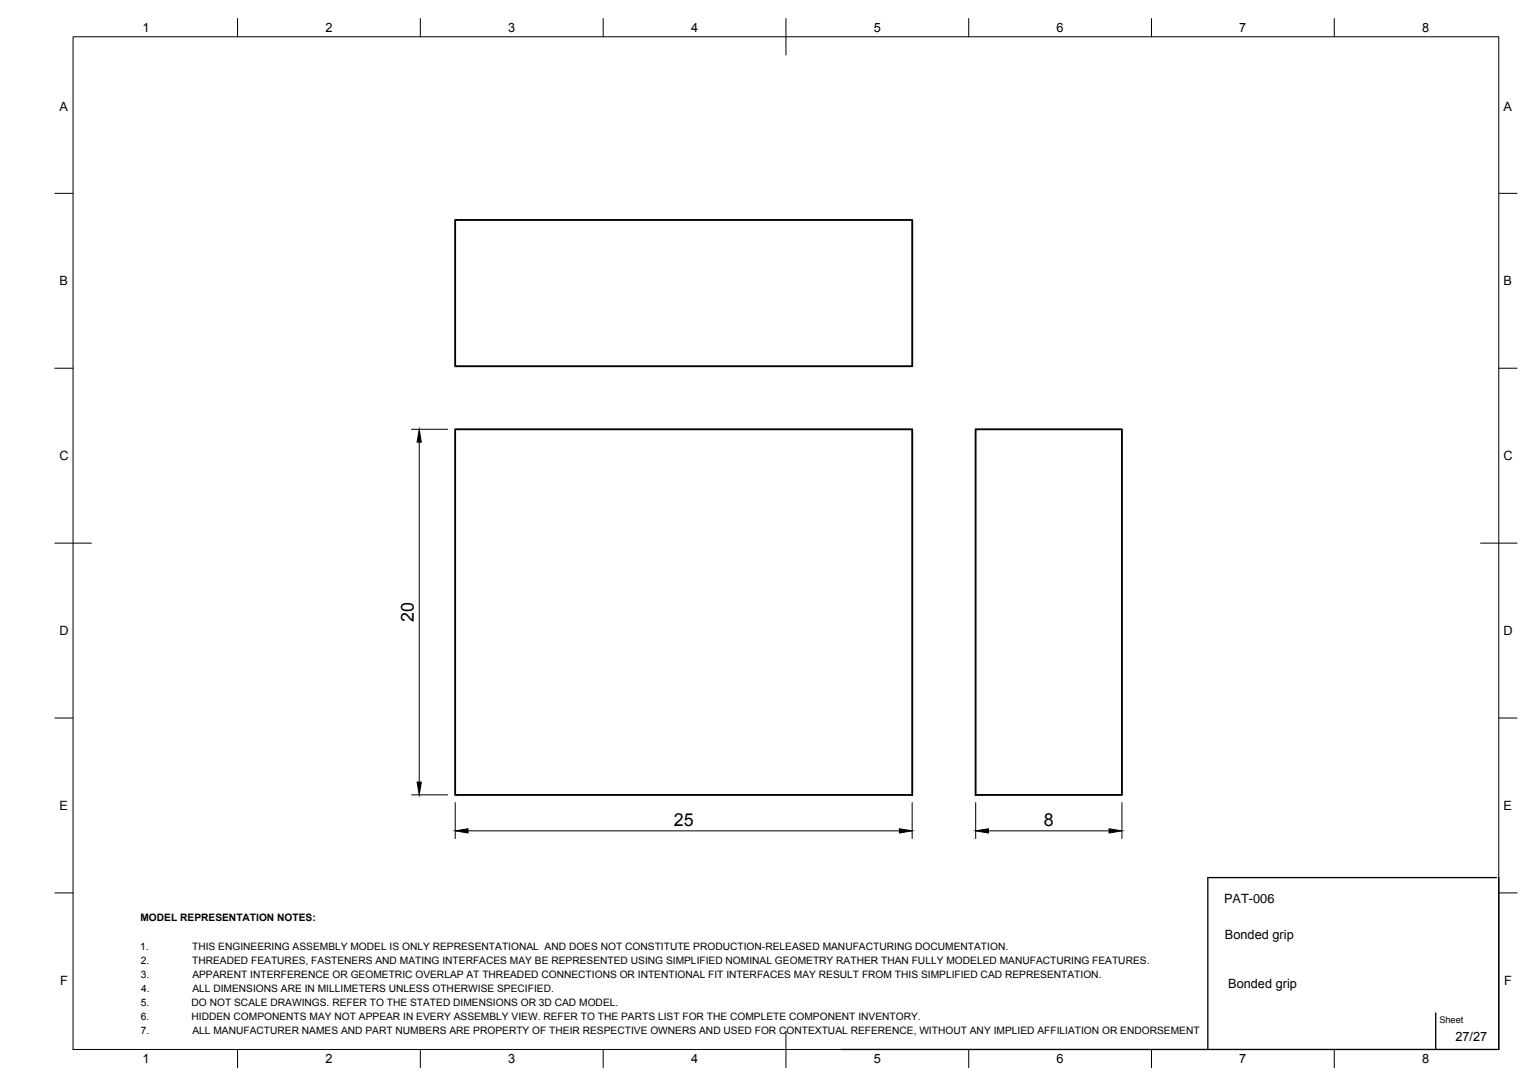
ISO-10303-21;
HEADER;
/* Generated by software containing ST-Developer
 * from STEP Tools, Inc. (www.steptools.com) 
 */

FILE_DESCRIPTION(
/* description */ ('Ball-type isolation valve (generic)'),
/* implementation_level */ '2;1');

FILE_NAME(
/* name */ 'Bonded grip.step',
/* time_stamp */ '2026-10-27T10:53:05-07:00',
/* author */ (''),
/* organization */ (''),
/* preprocessor_version */ 'ST-DEVELOPER v20.2',
/* originating_system */ 'Autodesk Translation Framework v15.17.0.0',
/* authorisation */ '');

FILE_SCHEMA (('AUTOMOTIVE_DESIGN { 1 0 10303 214 3 1 1 }'));
ENDSEC;

DATA;
#10=MECHANICAL_DESIGN_GEOMETRIC_PRESENTATION_REPRESENTATION('',(#301),#7425);
#249=SHAPE_REPRESENTATION_RELATIONSHIP('SRR','None',#7560,#275);
#275=ADVANCED_BREP_SHAPE_REPRESENTATION('',(#325),#7423);
#301=STYLED_ITEM('',(#7751),#325);
#325=MANIFOLD_SOLID_BREP('Body1',#4108);
#562=PLANE('',#4858);
#563=PLANE('',#4859);
#564=PLANE('',#4860);
#565=PLANE('',#4861);
#566=PLANE('',#4862);
#567=PLANE('',#4863);
#806=FACE_OUTER_BOUND('',#1142,.T.);
#807=FACE_OUTER_BOUND('',#1143,.T.);
#808=FACE_OUTER_BOUND('',#1144,.T.);
#809=FACE_OUTER_BOUND('',#1145,.T.);
#810=FACE_OUTER_BOUND('',#1146,.T.);
#811=FACE_OUTER_BOUND('',#1147,.T.);
#1142=EDGE_LOOP('',(#3681,#3682,#3683,#3684));
#1143=EDGE_LOOP('',(#3685,#3686,#3687,#3688));
#1144=EDGE_LOOP('',(#3689,#3690,#3691,#3692));
#1145=EDGE_LOOP('',(#3693,#3694,#3695,#3696));
#1146=EDGE_LOOP('',(#3697,#3698,#3699,#3700));
#1147=EDGE_LOOP('',(#3701,#3702,#3703,#3704));
#1438=LINE('',#7269,#1746);
#1439=LINE('',#7271,#1747);
#1440=LINE('',#7273,#1748);
#1441=LINE('',#7274,#1749);
#1442=LINE('',#7277,#1750);
#1443=LINE('',#7279,#1751);
#1444=LINE('',#7280,#1752);
#1445=LINE('',#7283,#1753);
#1446=LINE('',#7285,#1754);
#1447=LINE('',#7286,#1755);
#1448=LINE('',#7288,#1756);
#1449=LINE('',#7289,#1757);
#1746=VECTOR('',#6091,1.);
#1747=VECTOR('',#6092,1.);
#1748=VECTOR('',#6093,1.);
#1749=VECTOR('',#6094,1.);
#1750=VECTOR('',#6097,1.);
#1751=VECTOR('',#6098,1.);
#1752=VECTOR('',#6099,1.);
#1753=VECTOR('',#6102,1.);
#1754=VECTOR('',#6103,1.);
#1755=VECTOR('',#6104,1.);
#1756=VECTOR('',#6107,1.);
#1757=VECTOR('',#6108,1.);
#2253=VERTEX_POINT('',#7267);
#2254=VERTEX_POINT('',#7268);
#2255=VERTEX_POINT('',#7270);
#2256=VERTEX_POINT('',#7272);
#2257=VERTEX_POINT('',#7276);
#2258=VERTEX_POINT('',#7278);
#2259=VERTEX_POINT('',#7282);
#2260=VERTEX_POINT('',#7284);
#2733=EDGE_CURVE('',#2253,#2254,#1438,.T.);
#2734=EDGE_CURVE('',#2254,#2255,#1439,.T.);
#2735=EDGE_CURVE('',#2256,#2255,#1440,.T.);
#2736=EDGE_CURVE('',#2253,#2256,#1441,.T.);
#2737=EDGE_CURVE('',#2257,#2253,#1442,.T.);
#2738=EDGE_CURVE('',#2258,#2256,#1443,.T.);
#2739=EDGE_CURVE('',#2257,#2258,#1444,.T.);
#2740=EDGE_CURVE('',#2259,#2257,#1445,.T.);
#2741=EDGE_CURVE('',#2260,#2258,#1446,.T.);
#2742=EDGE_CURVE('',#2259,#2260,#1447,.T.);
#2743=EDGE_CURVE('',#2254,#2259,#1448,.T.);
#2744=EDGE_CURVE('',#2255,#2260,#1449,.T.);
#3681=ORIENTED_EDGE('',*,*,#2733,.T.);
#3682=ORIENTED_EDGE('',*,*,#2734,.T.);
#3683=ORIENTED_EDGE('',*,*,#2735,.F.);
#3684=ORIENTED_EDGE('',*,*,#2736,.F.);
#3685=ORIENTED_EDGE('',*,*,#2737,.T.);
#3686=ORIENTED_EDGE('',*,*,#2736,.T.);
#3687=ORIENTED_EDGE('',*,*,#2738,.F.);
#3688=ORIENTED_EDGE('',*,*,#2739,.F.);
#3689=ORIENTED_EDGE('',*,*,#2740,.T.);
#3690=ORIENTED_EDGE('',*,*,#2739,.T.);
#3691=ORIENTED_EDGE('',*,*,#2741,.F.);
#3692=ORIENTED_EDGE('',*,*,#2742,.F.);
#3693=ORIENTED_EDGE('',*,*,#2743,.T.);
#3694=ORIENTED_EDGE('',*,*,#2742,.T.);
#3695=ORIENTED_EDGE('',*,*,#2744,.F.);
#3696=ORIENTED_EDGE('',*,*,#2734,.F.);
#3697=ORIENTED_EDGE('',*,*,#2744,.T.);
#3698=ORIENTED_EDGE('',*,*,#2741,.T.);
#3699=ORIENTED_EDGE('',*,*,#2738,.T.);
#3700=ORIENTED_EDGE('',*,*,#2735,.T.);
#3701=ORIENTED_EDGE('',*,*,#2743,.F.);
#3702=ORIENTED_EDGE('',*,*,#2733,.F.);
#3703=ORIENTED_EDGE('',*,*,#2737,.F.);
#3704=ORIENTED_EDGE('',*,*,#2740,.F.);
#4060=ADVANCED_FACE('',(#806),#562,.T.);
#4061=ADVANCED_FACE('',(#807),#563,.T.);
#4062=ADVANCED_FACE('',(#808),#564,.T.);
#4063=ADVANCED_FACE('',(#809),#565,.T.);
#4064=ADVANCED_FACE('',(#810),#566,.T.);
#4065=ADVANCED_FACE('',(#811),#567,.F.);
#4108=CLOSED_SHELL('',(#4060,#4061,#4062,#4063,#4064,#4065));
#4857=AXIS2_PLACEMENT_3D('',#7265,#6087,#6088);
#4858=AXIS2_PLACEMENT_3D('',#7266,#6089,#6090);
#4859=AXIS2_PLACEMENT_3D('',#7275,#6095,#6096);
#4860=AXIS2_PLACEMENT_3D('',#7281,#6100,#6101);
#4861=AXIS2_PLACEMENT_3D('',#7287,#6105,#6106);
#4862=AXIS2_PLACEMENT_3D('',#7290,#6109,#6110);
#4863=AXIS2_PLACEMENT_3D('',#7291,#6111,#6112);
#6087=DIRECTION('axis',(0.,0.,1.));
#6088=DIRECTION('refdir',(1.,0.,0.));
#6089=DIRECTION('center_axis',(0.,1.,0.));
#6090=DIRECTION('ref_axis',(-1.,0.,0.));
#6091=DIRECTION('',(-1.,0.,0.));
#6092=DIRECTION('',(0.,0.,1.));
#6093=DIRECTION('',(-1.,0.,0.));
#6094=DIRECTION('',(0.,0.,1.));
#6095=DIRECTION('center_axis',(1.,0.,0.));
#6096=DIRECTION('ref_axis',(0.,1.,0.));
#6097=DIRECTION('',(0.,1.,0.));
#6098=DIRECTION('',(0.,1.,0.));
#6099=DIRECTION('',(0.,0.,1.));
#6100=DIRECTION('center_axis',(0.,-1.,0.));
#6101=DIRECTION('ref_axis',(1.,0.,0.));
#6102=DIRECTION('',(1.,0.,0.));
#6103=DIRECTION('',(1.,0.,0.));
#6104=DIRECTION('',(0.,0.,1.));
#6105=DIRECTION('center_axis',(-1.,0.,0.));
#6106=DIRECTION('ref_axis',(0.,-1.,0.));
#6107=DIRECTION('',(0.,-1.,0.));
#6108=DIRECTION('',(0.,-1.,0.));
#6109=DIRECTION('center_axis',(0.,0.,1.));
#6110=DIRECTION('ref_axis',(1.,0.,0.));
#6111=DIRECTION('center_axis',(0.,0.,1.));
#6112=DIRECTION('ref_axis',(1.,0.,0.));
#7265=CARTESIAN_POINT('',(0.,0.,0.));
#7266=CARTESIAN_POINT('Origin',(8.5,1.,9.4));
#7267=CARTESIAN_POINT('',(8.5,1.,9.4));
#7268=CARTESIAN_POINT('',(6.,1.,9.4));
#7269=CARTESIAN_POINT('',(8.5,1.,9.4));
#7270=CARTESIAN_POINT('',(6.,1.,10.2));
#7271=CARTESIAN_POINT('',(6.,1.,9.4));
#7272=CARTESIAN_POINT('',(8.5,1.,10.2));
#7273=CARTESIAN_POINT('',(8.5,1.,10.2));
#7274=CARTESIAN_POINT('',(8.5,1.,9.4));
#7275=CARTESIAN_POINT('Origin',(8.5,-1.,9.4));
#7276=CARTESIAN_POINT('',(8.5,-1.,9.4));
#7277=CARTESIAN_POINT('',(8.5,-1.,9.4));
#7278=CARTESIAN_POINT('',(8.5,-1.,10.2));
#7279=CARTESIAN_POINT('',(8.5,-1.,10.2));
#7280=CARTESIAN_POINT('',(8.5,-1.,9.4));
#7281=CARTESIAN_POINT('Origin',(6.,-1.,9.4));
#7282=CARTESIAN_POINT('',(6.,-1.,9.4));
#7283=CARTESIAN_POINT('',(6.,-1.,9.4));
#7284=CARTESIAN_POINT('',(6.,-1.,10.2));
#7285=CARTESIAN_POINT('',(6.,-1.,10.2));
#7286=CARTESIAN_POINT('',(6.,-1.,9.4));
#7287=CARTESIAN_POINT('Origin',(6.,1.,9.4));
#7288=CARTESIAN_POINT('',(6.,1.,9.4));
#7289=CARTESIAN_POINT('',(6.,1.,10.2));
#7290=CARTESIAN_POINT('Origin',(7.25,0.,10.2));
#7291=CARTESIAN_POINT('Origin',(7.25,0.,9.4));
#7393=UNCERTAINTY_MEASURE_WITH_UNIT(LENGTH_MEASURE(0.001),#7426,
'DISTANCE_ACCURACY_VALUE',
'Maximum model space distance between geometric entities at asserted c
onnectivities');
#7395=UNCERTAINTY_MEASURE_WITH_UNIT(LENGTH_MEASURE(0.001),#7426,
'DISTANCE_ACCURACY_VALUE',
'Maximum model space distance between geometric entities at asserted c
onnectivities');
#7423=(
GEOMETRIC_REPRESENTATION_CONTEXT(3)
GLOBAL_UNCERTAINTY_ASSIGNED_CONTEXT((#7393))
GLOBAL_UNIT_ASSIGNED_CONTEXT((#7426,#7428,#7429))
REPRESENTATION_CONTEXT('','3D')
);
#7425=(
GEOMETRIC_REPRESENTATION_CONTEXT(3)
GLOBAL_UNCERTAINTY_ASSIGNED_CONTEXT((#7395))
GLOBAL_UNIT_ASSIGNED_CONTEXT((#7426,#7428,#7429))
REPRESENTATION_CONTEXT('','3D')
);
#7426=(
LENGTH_UNIT()
NAMED_UNIT(*)
SI_UNIT(.CENTI.,.METRE.)
);
#7428=(
NAMED_UNIT(*)
PLANE_ANGLE_UNIT()
SI_UNIT($,.RADIAN.)
);
#7429=(
NAMED_UNIT(*)
SI_UNIT($,.STERADIAN.)
SOLID_ANGLE_UNIT()
);
#7457=SHAPE_DEFINITION_REPRESENTATION(#7523,#7560);
#7523=PRODUCT_DEFINITION_SHAPE('',$,#7590);
#7560=SHAPE_REPRESENTATION('',(#4857),#7423);
#7562=PRODUCT_DEFINITION_CONTEXT('part definition',#7651,'design');
#7590=PRODUCT_DEFINITION('Bonded grip','Bonded grip',#7619,#7562);
#7619=PRODUCT_DEFINITION_FORMATION('',$,#7680);
#7651=APPLICATION_CONTEXT(
'Core Data for Automotive Mechanical Design Process');
#7652=PRODUCT_CONTEXT('part definition',#7651,'mechanical');
#7680=PRODUCT('Bonded grip','Bonded grip','Bonded grip',(#7652));
#7745=COLOUR_RGB('Black',0.12,0.14,0.17);
#7746=FILL_AREA_STYLE_COLOUR('',#7745);
#7747=FILL_AREA_STYLE('',(#7746));
#7748=SURFACE_STYLE_FILL_AREA(#7747);
#7749=SURFACE_SIDE_STYLE('',(#7748));
#7750=SURFACE_STYLE_USAGE(.BOTH.,#7749);
#7751=PRESENTATION_STYLE_ASSIGNMENT((#7750));
ENDSEC;
END-ISO-10303-21;
